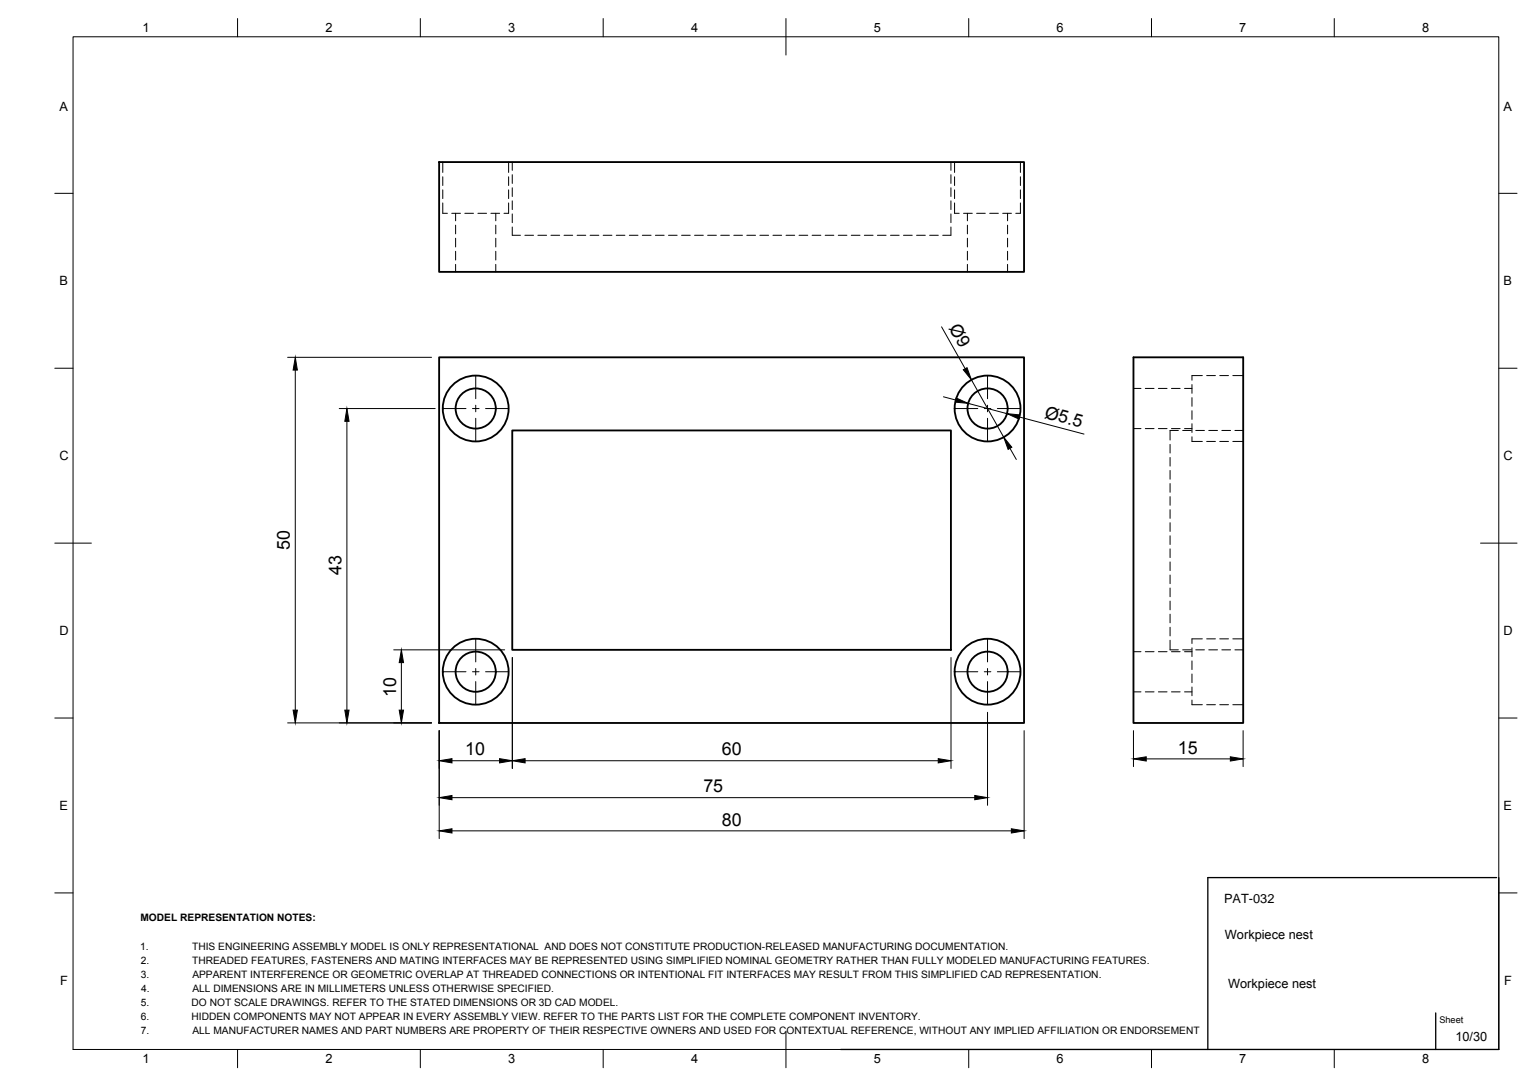
ISO-10303-21;
HEADER;
/* Generated by software containing ST-Developer
 * from STEP Tools, Inc. (www.steptools.com) 
 */

FILE_DESCRIPTION(
/* description */ ('Drill jig with bushing plate'),
/* implementation_level */ '2;1');

FILE_NAME(
/* name */ 'Workpiece nest.step',
/* time_stamp */ '2026-10-27T10:51:08-07:00',
/* author */ (''),
/* organization */ (''),
/* preprocessor_version */ 'ST-DEVELOPER v20.2',
/* originating_system */ 'Autodesk Translation Framework v15.17.0.0',
/* authorisation */ '');

FILE_SCHEMA (('AUTOMOTIVE_DESIGN { 1 0 10303 214 3 1 1 }'));
ENDSEC;

DATA;
#10=MECHANICAL_DESIGN_GEOMETRIC_PRESENTATION_REPRESENTATION('',(#228),#6638);
#180=SHAPE_REPRESENTATION_RELATIONSHIP('SRR','None',#6744,#204);
#204=ADVANCED_BREP_SHAPE_REPRESENTATION('',(#252),#6617);
#228=STYLED_ITEM('',(#6936),#252);
#252=MANIFOLD_SOLID_BREP('Body1',#3595);
#297=FACE_BOUND('',#777,.T.);
#298=FACE_BOUND('',#780,.T.);
#299=FACE_BOUND('',#783,.T.);
#300=FACE_BOUND('',#786,.T.);
#301=FACE_BOUND('',#801,.T.);
#302=FACE_BOUND('',#802,.T.);
#303=FACE_BOUND('',#803,.T.);
#304=FACE_BOUND('',#804,.T.);
#305=FACE_BOUND('',#805,.T.);
#306=FACE_BOUND('',#807,.T.);
#307=FACE_BOUND('',#808,.T.);
#308=FACE_BOUND('',#809,.T.);
#309=FACE_BOUND('',#810,.T.);
#384=PLANE('',#3960);
#385=PLANE('',#3965);
#386=PLANE('',#3970);
#387=PLANE('',#3975);
#388=PLANE('',#3985);
#389=PLANE('',#3986);
#390=PLANE('',#3987);
#391=PLANE('',#3988);
#392=PLANE('',#3989);
#393=PLANE('',#3990);
#394=PLANE('',#3991);
#395=PLANE('',#3992);
#396=PLANE('',#3993);
#397=PLANE('',#3994);
#398=PLANE('',#3995);
#533=FACE_OUTER_BOUND('',#775,.T.);
#534=FACE_OUTER_BOUND('',#776,.T.);
#535=FACE_OUTER_BOUND('',#778,.T.);
#536=FACE_OUTER_BOUND('',#779,.T.);
#537=FACE_OUTER_BOUND('',#781,.T.);
#538=FACE_OUTER_BOUND('',#782,.T.);
#539=FACE_OUTER_BOUND('',#784,.T.);
#540=FACE_OUTER_BOUND('',#785,.T.);
#541=FACE_OUTER_BOUND('',#787,.T.);
#542=FACE_OUTER_BOUND('',#788,.T.);
#543=FACE_OUTER_BOUND('',#789,.T.);
#544=FACE_OUTER_BOUND('',#790,.T.);
#545=FACE_OUTER_BOUND('',#791,.T.);
#546=FACE_OUTER_BOUND('',#792,.T.);
#547=FACE_OUTER_BOUND('',#793,.T.);
#548=FACE_OUTER_BOUND('',#794,.T.);
#549=FACE_OUTER_BOUND('',#795,.T.);
#550=FACE_OUTER_BOUND('',#796,.T.);
#551=FACE_OUTER_BOUND('',#797,.T.);
#552=FACE_OUTER_BOUND('',#798,.T.);
#553=FACE_OUTER_BOUND('',#799,.T.);
#554=FACE_OUTER_BOUND('',#800,.T.);
#555=FACE_OUTER_BOUND('',#806,.T.);
#775=EDGE_LOOP('',(#2569,#2570,#2571,#2572));
#776=EDGE_LOOP('',(#2573));
#777=EDGE_LOOP('',(#2574));
#778=EDGE_LOOP('',(#2575,#2576,#2577,#2578));
#779=EDGE_LOOP('',(#2579));
#780=EDGE_LOOP('',(#2580));
#781=EDGE_LOOP('',(#2581,#2582,#2583,#2584));
#782=EDGE_LOOP('',(#2585));
#783=EDGE_LOOP('',(#2586));
#784=EDGE_LOOP('',(#2587,#2588,#2589,#2590));
#785=EDGE_LOOP('',(#2591));
#786=EDGE_LOOP('',(#2592));
#787=EDGE_LOOP('',(#2593,#2594,#2595,#2596));
#788=EDGE_LOOP('',(#2597,#2598,#2599,#2600));
#789=EDGE_LOOP('',(#2601,#2602,#2603,#2604));
#790=EDGE_LOOP('',(#2605,#2606,#2607,#2608));
#791=EDGE_LOOP('',(#2609,#2610,#2611,#2612));
#792=EDGE_LOOP('',(#2613,#2614,#2615,#2616));
#793=EDGE_LOOP('',(#2617,#2618,#2619,#2620));
#794=EDGE_LOOP('',(#2621,#2622,#2623,#2624));
#795=EDGE_LOOP('',(#2625,#2626,#2627,#2628));
#796=EDGE_LOOP('',(#2629,#2630,#2631,#2632));
#797=EDGE_LOOP('',(#2633,#2634,#2635,#2636));
#798=EDGE_LOOP('',(#2637,#2638,#2639,#2640));
#799=EDGE_LOOP('',(#2641,#2642,#2643,#2644));
#800=EDGE_LOOP('',(#2645,#2646,#2647,#2648));
#801=EDGE_LOOP('',(#2649,#2650,#2651,#2652));
#802=EDGE_LOOP('',(#2653));
#803=EDGE_LOOP('',(#2654));
#804=EDGE_LOOP('',(#2655));
#805=EDGE_LOOP('',(#2656));
#806=EDGE_LOOP('',(#2657,#2658,#2659,#2660));
#807=EDGE_LOOP('',(#2661));
#808=EDGE_LOOP('',(#2662));
#809=EDGE_LOOP('',(#2663));
#810=EDGE_LOOP('',(#2664));
#1060=LINE('',#5640,#1321);
#1061=LINE('',#5649,#1322);
#1062=LINE('',#5658,#1323);
#1063=LINE('',#5667,#1324);
#1064=LINE('',#5675,#1325);
#1065=LINE('',#5679,#1326);
#1066=LINE('',#5683,#1327);
#1067=LINE('',#5687,#1328);
#1068=LINE('',#5691,#1329);
#1069=LINE('',#5693,#1330);
#1070=LINE('',#5695,#1331);
#1071=LINE('',#5696,#1332);
#1072=LINE('',#5699,#1333);
#1073=LINE('',#5701,#1334);
#1074=LINE('',#5702,#1335);
#1075=LINE('',#5705,#1336);
#1076=LINE('',#5707,#1337);
#1077=LINE('',#5708,#1338);
#1078=LINE('',#5710,#1339);
#1079=LINE('',#5711,#1340);
#1080=LINE('',#5716,#1341);
#1081=LINE('',#5718,#1342);
#1082=LINE('',#5720,#1343);
#1083=LINE('',#5721,#1344);
#1084=LINE('',#5724,#1345);
#1085=LINE('',#5726,#1346);
#1086=LINE('',#5727,#1347);
#1087=LINE('',#5730,#1348);
#1088=LINE('',#5732,#1349);
#1089=LINE('',#5733,#1350);
#1090=LINE('',#5735,#1351);
#1091=LINE('',#5736,#1352);
#1321=VECTOR('',#4515,0.45);
#1322=VECTOR('',#4526,0.45);
#1323=VECTOR('',#4537,0.45);
#1324=VECTOR('',#4548,0.45);
#1325=VECTOR('',#4559,0.275);
#1326=VECTOR('',#4564,0.275);
#1327=VECTOR('',#4569,0.275);
#1328=VECTOR('',#4574,0.275);
#1329=VECTOR('',#4577,1.);
#1330=VECTOR('',#4578,1.);
#1331=VECTOR('',#4579,1.);
#1332=VECTOR('',#4580,1.);
#1333=VECTOR('',#4583,1.);
#1334=VECTOR('',#4584,1.);
#1335=VECTOR('',#4585,1.);
#1336=VECTOR('',#4588,1.);
#1337=VECTOR('',#4589,1.);
#1338=VECTOR('',#4590,1.);
#1339=VECTOR('',#4593,1.);
#1340=VECTOR('',#4594,1.);
#1341=VECTOR('',#4599,1.);
#1342=VECTOR('',#4600,1.);
#1343=VECTOR('',#4601,1.);
#1344=VECTOR('',#4602,1.);
#1345=VECTOR('',#4605,1.);
#1346=VECTOR('',#4606,1.);
#1347=VECTOR('',#4607,1.);
#1348=VECTOR('',#4610,1.);
#1349=VECTOR('',#4611,1.);
#1350=VECTOR('',#4612,1.);
#1351=VECTOR('',#4615,1.);
#1352=VECTOR('',#4616,1.);
#1588=CIRCLE('',#3958,0.45);
#1589=CIRCLE('',#3959,0.45);
#1590=CIRCLE('',#3961,0.275);
#1591=CIRCLE('',#3963,0.45);
#1592=CIRCLE('',#3964,0.45);
#1593=CIRCLE('',#3966,0.275);
#1594=CIRCLE('',#3968,0.45);
#1595=CIRCLE('',#3969,0.45);
#1596=CIRCLE('',#3971,0.275);
#1597=CIRCLE('',#3973,0.45);
#1598=CIRCLE('',#3974,0.45);
#1599=CIRCLE('',#3976,0.275);
#1600=CIRCLE('',#3978,0.275);
#1601=CIRCLE('',#3980,0.275);
#1602=CIRCLE('',#3982,0.275);
#1603=CIRCLE('',#3984,0.275);
#1764=VERTEX_POINT('',#5637);
#1765=VERTEX_POINT('',#5639);
#1766=VERTEX_POINT('',#5643);
#1767=VERTEX_POINT('',#5646);
#1768=VERTEX_POINT('',#5648);
#1769=VERTEX_POINT('',#5652);
#1770=VERTEX_POINT('',#5655);
#1771=VERTEX_POINT('',#5657);
#1772=VERTEX_POINT('',#5661);
#1773=VERTEX_POINT('',#5664);
#1774=VERTEX_POINT('',#5666);
#1775=VERTEX_POINT('',#5670);
#1776=VERTEX_POINT('',#5673);
#1777=VERTEX_POINT('',#5677);
#1778=VERTEX_POINT('',#5681);
#1779=VERTEX_POINT('',#5685);
#1780=VERTEX_POINT('',#5689);
#1781=VERTEX_POINT('',#5690);
#1782=VERTEX_POINT('',#5692);
#1783=VERTEX_POINT('',#5694);
#1784=VERTEX_POINT('',#5698);
#1785=VERTEX_POINT('',#5700);
#1786=VERTEX_POINT('',#5704);
#1787=VERTEX_POINT('',#5706);
#1788=VERTEX_POINT('',#5714);
#1789=VERTEX_POINT('',#5715);
#1790=VERTEX_POINT('',#5717);
#1791=VERTEX_POINT('',#5719);
#1792=VERTEX_POINT('',#5723);
#1793=VERTEX_POINT('',#5725);
#1794=VERTEX_POINT('',#5729);
#1795=VERTEX_POINT('',#5731);
#2072=EDGE_CURVE('',#1764,#1764,#1588,.T.);
#2073=EDGE_CURVE('',#1764,#1765,#1060,.T.);
#2074=EDGE_CURVE('',#1765,#1765,#1589,.T.);
#2075=EDGE_CURVE('',#1766,#1766,#1590,.T.);
#2076=EDGE_CURVE('',#1767,#1767,#1591,.T.);
#2077=EDGE_CURVE('',#1767,#1768,#1061,.T.);
#2078=EDGE_CURVE('',#1768,#1768,#1592,.T.);
#2079=EDGE_CURVE('',#1769,#1769,#1593,.T.);
#2080=EDGE_CURVE('',#1770,#1770,#1594,.T.);
#2081=EDGE_CURVE('',#1770,#1771,#1062,.T.);
#2082=EDGE_CURVE('',#1771,#1771,#1595,.T.);
#2083=EDGE_CURVE('',#1772,#1772,#1596,.T.);
#2084=EDGE_CURVE('',#1773,#1773,#1597,.T.);
#2085=EDGE_CURVE('',#1773,#1774,#1063,.T.);
#2086=EDGE_CURVE('',#1774,#1774,#1598,.T.);
#2087=EDGE_CURVE('',#1775,#1775,#1599,.T.);
#2088=EDGE_CURVE('',#1776,#1776,#1600,.T.);
#2089=EDGE_CURVE('',#1776,#1766,#1064,.T.);
#2090=EDGE_CURVE('',#1777,#1777,#1601,.T.);
#2091=EDGE_CURVE('',#1777,#1769,#1065,.T.);
#2092=EDGE_CURVE('',#1778,#1778,#1602,.T.);
#2093=EDGE_CURVE('',#1778,#1772,#1066,.T.);
#2094=EDGE_CURVE('',#1779,#1779,#1603,.T.);
#2095=EDGE_CURVE('',#1779,#1775,#1067,.T.);
#2096=EDGE_CURVE('',#1780,#1781,#1068,.T.);
#2097=EDGE_CURVE('',#1782,#1780,#1069,.T.);
#2098=EDGE_CURVE('',#1783,#1782,#1070,.T.);
#2099=EDGE_CURVE('',#1783,#1781,#1071,.T.);
#2100=EDGE_CURVE('',#1781,#1784,#1072,.T.);
#2101=EDGE_CURVE('',#1785,#1783,#1073,.T.);
#2102=EDGE_CURVE('',#1785,#1784,#1074,.T.);
#2103=EDGE_CURVE('',#1784,#1786,#1075,.T.);
#2104=EDGE_CURVE('',#1787,#1785,#1076,.T.);
#2105=EDGE_CURVE('',#1787,#1786,#1077,.T.);
#2106=EDGE_CURVE('',#1786,#1780,#1078,.T.);
#2107=EDGE_CURVE('',#1782,#1787,#1079,.T.);
#2108=EDGE_CURVE('',#1788,#1789,#1080,.T.);
#2109=EDGE_CURVE('',#1789,#1790,#1081,.T.);
#2110=EDGE_CURVE('',#1791,#1790,#1082,.T.);
#2111=EDGE_CURVE('',#1788,#1791,#1083,.T.);
#2112=EDGE_CURVE('',#1792,#1788,#1084,.T.);
#2113=EDGE_CURVE('',#1793,#1791,#1085,.T.);
#2114=EDGE_CURVE('',#1792,#1793,#1086,.T.);
#2115=EDGE_CURVE('',#1794,#1792,#1087,.T.);
#2116=EDGE_CURVE('',#1795,#1793,#1088,.T.);
#2117=EDGE_CURVE('',#1794,#1795,#1089,.T.);
#2118=EDGE_CURVE('',#1789,#1794,#1090,.T.);
#2119=EDGE_CURVE('',#1790,#1795,#1091,.T.);
#2569=ORIENTED_EDGE('',*,*,#2072,.F.);
#2570=ORIENTED_EDGE('',*,*,#2073,.T.);
#2571=ORIENTED_EDGE('',*,*,#2074,.F.);
#2572=ORIENTED_EDGE('',*,*,#2073,.F.);
#2573=ORIENTED_EDGE('',*,*,#2072,.T.);
#2574=ORIENTED_EDGE('',*,*,#2075,.F.);
#2575=ORIENTED_EDGE('',*,*,#2076,.F.);
#2576=ORIENTED_EDGE('',*,*,#2077,.T.);
#2577=ORIENTED_EDGE('',*,*,#2078,.F.);
#2578=ORIENTED_EDGE('',*,*,#2077,.F.);
#2579=ORIENTED_EDGE('',*,*,#2076,.T.);
#2580=ORIENTED_EDGE('',*,*,#2079,.F.);
#2581=ORIENTED_EDGE('',*,*,#2080,.F.);
#2582=ORIENTED_EDGE('',*,*,#2081,.T.);
#2583=ORIENTED_EDGE('',*,*,#2082,.F.);
#2584=ORIENTED_EDGE('',*,*,#2081,.F.);
#2585=ORIENTED_EDGE('',*,*,#2080,.T.);
#2586=ORIENTED_EDGE('',*,*,#2083,.F.);
#2587=ORIENTED_EDGE('',*,*,#2084,.F.);
#2588=ORIENTED_EDGE('',*,*,#2085,.T.);
#2589=ORIENTED_EDGE('',*,*,#2086,.F.);
#2590=ORIENTED_EDGE('',*,*,#2085,.F.);
#2591=ORIENTED_EDGE('',*,*,#2084,.T.);
#2592=ORIENTED_EDGE('',*,*,#2087,.F.);
#2593=ORIENTED_EDGE('',*,*,#2088,.F.);
#2594=ORIENTED_EDGE('',*,*,#2089,.T.);
#2595=ORIENTED_EDGE('',*,*,#2075,.T.);
#2596=ORIENTED_EDGE('',*,*,#2089,.F.);
#2597=ORIENTED_EDGE('',*,*,#2090,.F.);
#2598=ORIENTED_EDGE('',*,*,#2091,.T.);
#2599=ORIENTED_EDGE('',*,*,#2079,.T.);
#2600=ORIENTED_EDGE('',*,*,#2091,.F.);
#2601=ORIENTED_EDGE('',*,*,#2092,.F.);
#2602=ORIENTED_EDGE('',*,*,#2093,.T.);
#2603=ORIENTED_EDGE('',*,*,#2083,.T.);
#2604=ORIENTED_EDGE('',*,*,#2093,.F.);
#2605=ORIENTED_EDGE('',*,*,#2094,.F.);
#2606=ORIENTED_EDGE('',*,*,#2095,.T.);
#2607=ORIENTED_EDGE('',*,*,#2087,.T.);
#2608=ORIENTED_EDGE('',*,*,#2095,.F.);
#2609=ORIENTED_EDGE('',*,*,#2096,.F.);
#2610=ORIENTED_EDGE('',*,*,#2097,.F.);
#2611=ORIENTED_EDGE('',*,*,#2098,.F.);
#2612=ORIENTED_EDGE('',*,*,#2099,.T.);
#2613=ORIENTED_EDGE('',*,*,#2100,.F.);
#2614=ORIENTED_EDGE('',*,*,#2099,.F.);
#2615=ORIENTED_EDGE('',*,*,#2101,.F.);
#2616=ORIENTED_EDGE('',*,*,#2102,.T.);
#2617=ORIENTED_EDGE('',*,*,#2103,.F.);
#2618=ORIENTED_EDGE('',*,*,#2102,.F.);
#2619=ORIENTED_EDGE('',*,*,#2104,.F.);
#2620=ORIENTED_EDGE('',*,*,#2105,.T.);
#2621=ORIENTED_EDGE('',*,*,#2106,.F.);
#2622=ORIENTED_EDGE('',*,*,#2105,.F.);
#2623=ORIENTED_EDGE('',*,*,#2107,.F.);
#2624=ORIENTED_EDGE('',*,*,#2097,.T.);
#2625=ORIENTED_EDGE('',*,*,#2101,.T.);
#2626=ORIENTED_EDGE('',*,*,#2098,.T.);
#2627=ORIENTED_EDGE('',*,*,#2107,.T.);
#2628=ORIENTED_EDGE('',*,*,#2104,.T.);
#2629=ORIENTED_EDGE('',*,*,#2108,.T.);
#2630=ORIENTED_EDGE('',*,*,#2109,.T.);
#2631=ORIENTED_EDGE('',*,*,#2110,.F.);
#2632=ORIENTED_EDGE('',*,*,#2111,.F.);
#2633=ORIENTED_EDGE('',*,*,#2112,.T.);
#2634=ORIENTED_EDGE('',*,*,#2111,.T.);
#2635=ORIENTED_EDGE('',*,*,#2113,.F.);
#2636=ORIENTED_EDGE('',*,*,#2114,.F.);
#2637=ORIENTED_EDGE('',*,*,#2115,.T.);
#2638=ORIENTED_EDGE('',*,*,#2114,.T.);
#2639=ORIENTED_EDGE('',*,*,#2116,.F.);
#2640=ORIENTED_EDGE('',*,*,#2117,.F.);
#2641=ORIENTED_EDGE('',*,*,#2118,.T.);
#2642=ORIENTED_EDGE('',*,*,#2117,.T.);
#2643=ORIENTED_EDGE('',*,*,#2119,.F.);
#2644=ORIENTED_EDGE('',*,*,#2109,.F.);
#2645=ORIENTED_EDGE('',*,*,#2119,.T.);
#2646=ORIENTED_EDGE('',*,*,#2116,.T.);
#2647=ORIENTED_EDGE('',*,*,#2113,.T.);
#2648=ORIENTED_EDGE('',*,*,#2110,.T.);
#2649=ORIENTED_EDGE('',*,*,#2103,.T.);
#2650=ORIENTED_EDGE('',*,*,#2106,.T.);
#2651=ORIENTED_EDGE('',*,*,#2096,.T.);
#2652=ORIENTED_EDGE('',*,*,#2100,.T.);
#2653=ORIENTED_EDGE('',*,*,#2086,.T.);
#2654=ORIENTED_EDGE('',*,*,#2082,.T.);
#2655=ORIENTED_EDGE('',*,*,#2078,.T.);
#2656=ORIENTED_EDGE('',*,*,#2074,.T.);
#2657=ORIENTED_EDGE('',*,*,#2118,.F.);
#2658=ORIENTED_EDGE('',*,*,#2108,.F.);
#2659=ORIENTED_EDGE('',*,*,#2112,.F.);
#2660=ORIENTED_EDGE('',*,*,#2115,.F.);
#2661=ORIENTED_EDGE('',*,*,#2088,.T.);
#2662=ORIENTED_EDGE('',*,*,#2090,.T.);
#2663=ORIENTED_EDGE('',*,*,#2092,.T.);
#2664=ORIENTED_EDGE('',*,*,#2094,.T.);
#3317=CYLINDRICAL_SURFACE('',#3957,0.45);
#3318=CYLINDRICAL_SURFACE('',#3962,0.45);
#3319=CYLINDRICAL_SURFACE('',#3967,0.45);
#3320=CYLINDRICAL_SURFACE('',#3972,0.45);
#3321=CYLINDRICAL_SURFACE('',#3977,0.275);
#3322=CYLINDRICAL_SURFACE('',#3979,0.275);
#3323=CYLINDRICAL_SURFACE('',#3981,0.275);
#3324=CYLINDRICAL_SURFACE('',#3983,0.275);
#3408=ADVANCED_FACE('',(#533),#3317,.F.);
#3409=ADVANCED_FACE('',(#534,#297),#384,.T.);
#3410=ADVANCED_FACE('',(#535),#3318,.F.);
#3411=ADVANCED_FACE('',(#536,#298),#385,.T.);
#3412=ADVANCED_FACE('',(#537),#3319,.F.);
#3413=ADVANCED_FACE('',(#538,#299),#386,.T.);
#3414=ADVANCED_FACE('',(#539),#3320,.F.);
#3415=ADVANCED_FACE('',(#540,#300),#387,.T.);
#3416=ADVANCED_FACE('',(#541),#3321,.F.);
#3417=ADVANCED_FACE('',(#542),#3322,.F.);
#3418=ADVANCED_FACE('',(#543),#3323,.F.);
#3419=ADVANCED_FACE('',(#544),#3324,.F.);
#3420=ADVANCED_FACE('',(#545),#388,.F.);
#3421=ADVANCED_FACE('',(#546),#389,.F.);
#3422=ADVANCED_FACE('',(#547),#390,.F.);
#3423=ADVANCED_FACE('',(#548),#391,.F.);
#3424=ADVANCED_FACE('',(#549),#392,.T.);
#3425=ADVANCED_FACE('',(#550),#393,.T.);
#3426=ADVANCED_FACE('',(#551),#394,.T.);
#3427=ADVANCED_FACE('',(#552),#395,.T.);
#3428=ADVANCED_FACE('',(#553),#396,.T.);
#3429=ADVANCED_FACE('',(#554,#301,#302,#303,#304,#305),#397,.T.);
#3430=ADVANCED_FACE('',(#555,#306,#307,#308,#309),#398,.F.);
#3595=CLOSED_SHELL('',(#3408,#3409,#3410,#3411,#3412,#3413,#3414,#3415,
#3416,#3417,#3418,#3419,#3420,#3421,#3422,#3423,#3424,#3425,#3426,#3427,
#3428,#3429,#3430));
#3956=AXIS2_PLACEMENT_3D('',#5635,#4509,#4510);
#3957=AXIS2_PLACEMENT_3D('',#5636,#4511,#4512);
#3958=AXIS2_PLACEMENT_3D('',#5638,#4513,#4514);
#3959=AXIS2_PLACEMENT_3D('',#5641,#4516,#4517);
#3960=AXIS2_PLACEMENT_3D('',#5642,#4518,#4519);
#3961=AXIS2_PLACEMENT_3D('',#5644,#4520,#4521);
#3962=AXIS2_PLACEMENT_3D('',#5645,#4522,#4523);
#3963=AXIS2_PLACEMENT_3D('',#5647,#4524,#4525);
#3964=AXIS2_PLACEMENT_3D('',#5650,#4527,#4528);
#3965=AXIS2_PLACEMENT_3D('',#5651,#4529,#4530);
#3966=AXIS2_PLACEMENT_3D('',#5653,#4531,#4532);
#3967=AXIS2_PLACEMENT_3D('',#5654,#4533,#4534);
#3968=AXIS2_PLACEMENT_3D('',#5656,#4535,#4536);
#3969=AXIS2_PLACEMENT_3D('',#5659,#4538,#4539);
#3970=AXIS2_PLACEMENT_3D('',#5660,#4540,#4541);
#3971=AXIS2_PLACEMENT_3D('',#5662,#4542,#4543);
#3972=AXIS2_PLACEMENT_3D('',#5663,#4544,#4545);
#3973=AXIS2_PLACEMENT_3D('',#5665,#4546,#4547);
#3974=AXIS2_PLACEMENT_3D('',#5668,#4549,#4550);
#3975=AXIS2_PLACEMENT_3D('',#5669,#4551,#4552);
#3976=AXIS2_PLACEMENT_3D('',#5671,#4553,#4554);
#3977=AXIS2_PLACEMENT_3D('',#5672,#4555,#4556);
#3978=AXIS2_PLACEMENT_3D('',#5674,#4557,#4558);
#3979=AXIS2_PLACEMENT_3D('',#5676,#4560,#4561);
#3980=AXIS2_PLACEMENT_3D('',#5678,#4562,#4563);
#3981=AXIS2_PLACEMENT_3D('',#5680,#4565,#4566);
#3982=AXIS2_PLACEMENT_3D('',#5682,#4567,#4568);
#3983=AXIS2_PLACEMENT_3D('',#5684,#4570,#4571);
#3984=AXIS2_PLACEMENT_3D('',#5686,#4572,#4573);
#3985=AXIS2_PLACEMENT_3D('',#5688,#4575,#4576);
#3986=AXIS2_PLACEMENT_3D('',#5697,#4581,#4582);
#3987=AXIS2_PLACEMENT_3D('',#5703,#4586,#4587);
#3988=AXIS2_PLACEMENT_3D('',#5709,#4591,#4592);
#3989=AXIS2_PLACEMENT_3D('',#5712,#4595,#4596);
#3990=AXIS2_PLACEMENT_3D('',#5713,#4597,#4598);
#3991=AXIS2_PLACEMENT_3D('',#5722,#4603,#4604);
#3992=AXIS2_PLACEMENT_3D('',#5728,#4608,#4609);
#3993=AXIS2_PLACEMENT_3D('',#5734,#4613,#4614);
#3994=AXIS2_PLACEMENT_3D('',#5737,#4617,#4618);
#3995=AXIS2_PLACEMENT_3D('',#5738,#4619,#4620);
#4509=DIRECTION('axis',(0.,0.,1.));
#4510=DIRECTION('refdir',(1.,0.,0.));
#4511=DIRECTION('center_axis',(0.,0.,1.));
#4512=DIRECTION('ref_axis',(1.,0.,0.));
#4513=DIRECTION('center_axis',(0.,0.,1.));
#4514=DIRECTION('ref_axis',(1.,0.,0.));
#4515=DIRECTION('',(0.,0.,1.));
#4516=DIRECTION('center_axis',(0.,0.,-1.));
#4517=DIRECTION('ref_axis',(1.,0.,0.));
#4518=DIRECTION('center_axis',(0.,0.,1.));
#4519=DIRECTION('ref_axis',(1.,0.,0.));
#4520=DIRECTION('center_axis',(0.,0.,1.));
#4521=DIRECTION('ref_axis',(1.,0.,0.));
#4522=DIRECTION('center_axis',(0.,0.,1.));
#4523=DIRECTION('ref_axis',(1.,0.,0.));
#4524=DIRECTION('center_axis',(0.,0.,1.));
#4525=DIRECTION('ref_axis',(1.,0.,0.));
#4526=DIRECTION('',(0.,0.,1.));
#4527=DIRECTION('center_axis',(0.,0.,-1.));
#4528=DIRECTION('ref_axis',(1.,0.,0.));
#4529=DIRECTION('center_axis',(0.,0.,1.));
#4530=DIRECTION('ref_axis',(1.,0.,0.));
#4531=DIRECTION('center_axis',(0.,0.,1.));
#4532=DIRECTION('ref_axis',(1.,0.,0.));
#4533=DIRECTION('center_axis',(0.,0.,1.));
#4534=DIRECTION('ref_axis',(1.,0.,0.));
#4535=DIRECTION('center_axis',(0.,0.,1.));
#4536=DIRECTION('ref_axis',(1.,0.,0.));
#4537=DIRECTION('',(0.,0.,1.));
#4538=DIRECTION('center_axis',(0.,0.,-1.));
#4539=DIRECTION('ref_axis',(1.,0.,0.));
#4540=DIRECTION('center_axis',(0.,0.,1.));
#4541=DIRECTION('ref_axis',(1.,0.,0.));
#4542=DIRECTION('center_axis',(0.,0.,1.));
#4543=DIRECTION('ref_axis',(1.,0.,0.));
#4544=DIRECTION('center_axis',(0.,0.,1.));
#4545=DIRECTION('ref_axis',(1.,0.,0.));
#4546=DIRECTION('center_axis',(0.,0.,1.));
#4547=DIRECTION('ref_axis',(1.,0.,0.));
#4548=DIRECTION('',(0.,0.,1.));
#4549=DIRECTION('center_axis',(0.,0.,-1.));
#4550=DIRECTION('ref_axis',(1.,0.,0.));
#4551=DIRECTION('center_axis',(0.,0.,1.));
#4552=DIRECTION('ref_axis',(1.,0.,0.));
#4553=DIRECTION('center_axis',(0.,0.,1.));
#4554=DIRECTION('ref_axis',(1.,0.,0.));
#4555=DIRECTION('center_axis',(0.,0.,1.));
#4556=DIRECTION('ref_axis',(1.,0.,0.));
#4557=DIRECTION('center_axis',(0.,0.,1.));
#4558=DIRECTION('ref_axis',(1.,0.,0.));
#4559=DIRECTION('',(0.,0.,1.));
#4560=DIRECTION('center_axis',(0.,0.,1.));
#4561=DIRECTION('ref_axis',(1.,0.,0.));
#4562=DIRECTION('center_axis',(0.,0.,1.));
#4563=DIRECTION('ref_axis',(1.,0.,0.));
#4564=DIRECTION('',(0.,0.,1.));
#4565=DIRECTION('center_axis',(0.,0.,1.));
#4566=DIRECTION('ref_axis',(1.,0.,0.));
#4567=DIRECTION('center_axis',(0.,0.,1.));
#4568=DIRECTION('ref_axis',(1.,0.,0.));
#4569=DIRECTION('',(0.,0.,1.));
#4570=DIRECTION('center_axis',(0.,0.,1.));
#4571=DIRECTION('ref_axis',(1.,0.,0.));
#4572=DIRECTION('center_axis',(0.,0.,1.));
#4573=DIRECTION('ref_axis',(1.,0.,0.));
#4574=DIRECTION('',(0.,0.,1.));
#4575=DIRECTION('center_axis',(0.,-1.,0.));
#4576=DIRECTION('ref_axis',(1.,0.,0.));
#4577=DIRECTION('',(-1.,0.,0.));
#4578=DIRECTION('',(0.,0.,1.));
#4579=DIRECTION('',(1.,0.,0.));
#4580=DIRECTION('',(0.,0.,1.));
#4581=DIRECTION('center_axis',(-1.,0.,0.));
#4582=DIRECTION('ref_axis',(0.,-1.,0.));
#4583=DIRECTION('',(0.,1.,0.));
#4584=DIRECTION('',(0.,-1.,0.));
#4585=DIRECTION('',(0.,0.,1.));
#4586=DIRECTION('center_axis',(0.,1.,0.));
#4587=DIRECTION('ref_axis',(-1.,0.,0.));
#4588=DIRECTION('',(1.,0.,0.));
#4589=DIRECTION('',(-1.,0.,0.));
#4590=DIRECTION('',(0.,0.,1.));
#4591=DIRECTION('center_axis',(1.,0.,0.));
#4592=DIRECTION('ref_axis',(0.,1.,0.));
#4593=DIRECTION('',(0.,-1.,0.));
#4594=DIRECTION('',(0.,1.,0.));
#4595=DIRECTION('center_axis',(0.,0.,1.));
#4596=DIRECTION('ref_axis',(1.,0.,0.));
#4597=DIRECTION('center_axis',(0.,1.,0.));
#4598=DIRECTION('ref_axis',(-1.,0.,0.));
#4599=DIRECTION('',(-1.,0.,0.));
#4600=DIRECTION('',(0.,0.,1.));
#4601=DIRECTION('',(-1.,0.,0.));
#4602=DIRECTION('',(0.,0.,1.));
#4603=DIRECTION('center_axis',(1.,0.,0.));
#4604=DIRECTION('ref_axis',(0.,1.,0.));
#4605=DIRECTION('',(0.,1.,0.));
#4606=DIRECTION('',(0.,1.,0.));
#4607=DIRECTION('',(0.,0.,1.));
#4608=DIRECTION('center_axis',(0.,-1.,0.));
#4609=DIRECTION('ref_axis',(1.,0.,0.));
#4610=DIRECTION('',(1.,0.,0.));
#4611=DIRECTION('',(1.,0.,0.));
#4612=DIRECTION('',(0.,0.,1.));
#4613=DIRECTION('center_axis',(-1.,0.,0.));
#4614=DIRECTION('ref_axis',(0.,-1.,0.));
#4615=DIRECTION('',(0.,-1.,0.));
#4616=DIRECTION('',(0.,-1.,0.));
#4617=DIRECTION('center_axis',(0.,0.,1.));
#4618=DIRECTION('ref_axis',(1.,0.,0.));
#4619=DIRECTION('center_axis',(0.,0.,1.));
#4620=DIRECTION('ref_axis',(1.,0.,0.));
#5635=CARTESIAN_POINT('',(0.,0.,0.));
#5636=CARTESIAN_POINT('Origin',(3.5,-1.8,1.8));
#5637=CARTESIAN_POINT('',(3.05,-1.8,1.8));
#5638=CARTESIAN_POINT('Origin',(3.5,-1.8,1.8));
#5639=CARTESIAN_POINT('',(3.05,-1.8,2.5));
#5640=CARTESIAN_POINT('',(3.05,-1.8,1.8));
#5641=CARTESIAN_POINT('Origin',(3.5,-1.8,2.5));
#5642=CARTESIAN_POINT('Origin',(3.5,-1.8,1.8));
#5643=CARTESIAN_POINT('',(3.225,-1.8,1.8));
#5644=CARTESIAN_POINT('Origin',(3.5,-1.8,1.8));
#5645=CARTESIAN_POINT('Origin',(-3.5,1.8,1.8));
#5646=CARTESIAN_POINT('',(-3.95,1.8,1.8));
#5647=CARTESIAN_POINT('Origin',(-3.5,1.8,1.8));
#5648=CARTESIAN_POINT('',(-3.95,1.8,2.5));
#5649=CARTESIAN_POINT('',(-3.95,1.8,1.8));
#5650=CARTESIAN_POINT('Origin',(-3.5,1.8,2.5));
#5651=CARTESIAN_POINT('Origin',(-3.5,1.8,1.8));
#5652=CARTESIAN_POINT('',(-3.775,1.8,1.8));
#5653=CARTESIAN_POINT('Origin',(-3.5,1.8,1.8));
#5654=CARTESIAN_POINT('Origin',(-3.5,-1.8,1.8));
#5655=CARTESIAN_POINT('',(-3.95,-1.8,1.8));
#5656=CARTESIAN_POINT('Origin',(-3.5,-1.8,1.8));
#5657=CARTESIAN_POINT('',(-3.95,-1.8,2.5));
#5658=CARTESIAN_POINT('',(-3.95,-1.8,1.8));
#5659=CARTESIAN_POINT('Origin',(-3.5,-1.8,2.5));
#5660=CARTESIAN_POINT('Origin',(-3.5,-1.8,1.8));
#5661=CARTESIAN_POINT('',(-3.775,-1.8,1.8));
#5662=CARTESIAN_POINT('Origin',(-3.5,-1.8,1.8));
#5663=CARTESIAN_POINT('Origin',(3.5,1.8,1.8));
#5664=CARTESIAN_POINT('',(3.05,1.8,1.8));
#5665=CARTESIAN_POINT('Origin',(3.5,1.8,1.8));
#5666=CARTESIAN_POINT('',(3.05,1.8,2.5));
#5667=CARTESIAN_POINT('',(3.05,1.8,1.8));
#5668=CARTESIAN_POINT('Origin',(3.5,1.8,2.5));
#5669=CARTESIAN_POINT('Origin',(3.5,1.8,1.8));
#5670=CARTESIAN_POINT('',(3.225,1.8,1.8));
#5671=CARTESIAN_POINT('Origin',(3.5,1.8,1.8));
#5672=CARTESIAN_POINT('Origin',(3.5,-1.8,0.9));
#5673=CARTESIAN_POINT('',(3.225,-1.8,1.));
#5674=CARTESIAN_POINT('Origin',(3.5,-1.8,1.));
#5675=CARTESIAN_POINT('',(3.225,-1.8,0.9));
#5676=CARTESIAN_POINT('Origin',(-3.5,1.8,0.9));
#5677=CARTESIAN_POINT('',(-3.775,1.8,1.));
#5678=CARTESIAN_POINT('Origin',(-3.5,1.8,1.));
#5679=CARTESIAN_POINT('',(-3.775,1.8,0.9));
#5680=CARTESIAN_POINT('Origin',(-3.5,-1.8,0.9));
#5681=CARTESIAN_POINT('',(-3.775,-1.8,1.));
#5682=CARTESIAN_POINT('Origin',(-3.5,-1.8,1.));
#5683=CARTESIAN_POINT('',(-3.775,-1.8,0.9));
#5684=CARTESIAN_POINT('Origin',(3.5,1.8,0.9));
#5685=CARTESIAN_POINT('',(3.225,1.8,1.));
#5686=CARTESIAN_POINT('Origin',(3.5,1.8,1.));
#5687=CARTESIAN_POINT('',(3.225,1.8,0.9));
#5688=CARTESIAN_POINT('Origin',(-3.,-1.5,1.5));
#5689=CARTESIAN_POINT('',(3.,-1.5,2.5));
#5690=CARTESIAN_POINT('',(-3.,-1.5,2.5));
#5691=CARTESIAN_POINT('',(-1.5,-1.5,2.5));
#5692=CARTESIAN_POINT('',(3.,-1.5,1.5));
#5693=CARTESIAN_POINT('',(3.,-1.5,1.5));
#5694=CARTESIAN_POINT('',(-3.,-1.5,1.5));
#5695=CARTESIAN_POINT('',(-3.,-1.5,1.5));
#5696=CARTESIAN_POINT('',(-3.,-1.5,1.5));
#5697=CARTESIAN_POINT('Origin',(-3.,1.5,1.5));
#5698=CARTESIAN_POINT('',(-3.,1.5,2.5));
#5699=CARTESIAN_POINT('',(-3.,0.75,2.5));
#5700=CARTESIAN_POINT('',(-3.,1.5,1.5));
#5701=CARTESIAN_POINT('',(-3.,1.5,1.5));
#5702=CARTESIAN_POINT('',(-3.,1.5,1.5));
#5703=CARTESIAN_POINT('Origin',(3.,1.5,1.5));
#5704=CARTESIAN_POINT('',(3.,1.5,2.5));
#5705=CARTESIAN_POINT('',(1.5,1.5,2.5));
#5706=CARTESIAN_POINT('',(3.,1.5,1.5));
#5707=CARTESIAN_POINT('',(3.,1.5,1.5));
#5708=CARTESIAN_POINT('',(3.,1.5,1.5));
#5709=CARTESIAN_POINT('Origin',(3.,-1.5,1.5));
#5710=CARTESIAN_POINT('',(3.,-0.75,2.5));
#5711=CARTESIAN_POINT('',(3.,-1.5,1.5));
#5712=CARTESIAN_POINT('Origin',(0.,0.,1.5));
#5713=CARTESIAN_POINT('Origin',(4.,2.5,1.));
#5714=CARTESIAN_POINT('',(4.,2.5,1.));
#5715=CARTESIAN_POINT('',(-4.,2.5,1.));
#5716=CARTESIAN_POINT('',(4.,2.5,1.));
#5717=CARTESIAN_POINT('',(-4.,2.5,2.5));
#5718=CARTESIAN_POINT('',(-4.,2.5,1.));
#5719=CARTESIAN_POINT('',(4.,2.5,2.5));
#5720=CARTESIAN_POINT('',(4.,2.5,2.5));
#5721=CARTESIAN_POINT('',(4.,2.5,1.));
#5722=CARTESIAN_POINT('Origin',(4.,-2.5,1.));
#5723=CARTESIAN_POINT('',(4.,-2.5,1.));
#5724=CARTESIAN_POINT('',(4.,-2.5,1.));
#5725=CARTESIAN_POINT('',(4.,-2.5,2.5));
#5726=CARTESIAN_POINT('',(4.,-2.5,2.5));
#5727=CARTESIAN_POINT('',(4.,-2.5,1.));
#5728=CARTESIAN_POINT('Origin',(-4.,-2.5,1.));
#5729=CARTESIAN_POINT('',(-4.,-2.5,1.));
#5730=CARTESIAN_POINT('',(-4.,-2.5,1.));
#5731=CARTESIAN_POINT('',(-4.,-2.5,2.5));
#5732=CARTESIAN_POINT('',(-4.,-2.5,2.5));
#5733=CARTESIAN_POINT('',(-4.,-2.5,1.));
#5734=CARTESIAN_POINT('Origin',(-4.,2.5,1.));
#5735=CARTESIAN_POINT('',(-4.,2.5,1.));
#5736=CARTESIAN_POINT('',(-4.,2.5,2.5));
#5737=CARTESIAN_POINT('Origin',(0.,0.,2.5));
#5738=CARTESIAN_POINT('Origin',(0.,0.,1.));
#6588=UNCERTAINTY_MEASURE_WITH_UNIT(LENGTH_MEASURE(0.001),#6639,
'DISTANCE_ACCURACY_VALUE',
'Maximum model space distance between geometric entities at asserted c
onnectivities');
#6609=UNCERTAINTY_MEASURE_WITH_UNIT(LENGTH_MEASURE(0.001),#6639,
'DISTANCE_ACCURACY_VALUE',
'Maximum model space distance between geometric entities at asserted c
onnectivities');
#6617=(
GEOMETRIC_REPRESENTATION_CONTEXT(3)
GLOBAL_UNCERTAINTY_ASSIGNED_CONTEXT((#6588))
GLOBAL_UNIT_ASSIGNED_CONTEXT((#6639,#6641,#6642))
REPRESENTATION_CONTEXT('','3D')
);
#6638=(
GEOMETRIC_REPRESENTATION_CONTEXT(3)
GLOBAL_UNCERTAINTY_ASSIGNED_CONTEXT((#6609))
GLOBAL_UNIT_ASSIGNED_CONTEXT((#6639,#6641,#6642))
REPRESENTATION_CONTEXT('','3D')
);
#6639=(
LENGTH_UNIT()
NAMED_UNIT(*)
SI_UNIT(.CENTI.,.METRE.)
);
#6641=(
NAMED_UNIT(*)
PLANE_ANGLE_UNIT()
SI_UNIT($,.RADIAN.)
);
#6642=(
NAMED_UNIT(*)
SI_UNIT($,.STERADIAN.)
SOLID_ANGLE_UNIT()
);
#6650=SHAPE_DEFINITION_REPRESENTATION(#6678,#6744);
#6678=PRODUCT_DEFINITION_SHAPE('',$,#6773);
#6744=SHAPE_REPRESENTATION('',(#3956),#6617);
#6765=PRODUCT_DEFINITION_CONTEXT('part definition',#6851,'design');
#6773=PRODUCT_DEFINITION('Workpiece nest','Workpiece nest',#6801,#6765);
#6801=PRODUCT_DEFINITION_FORMATION('',$,#6860);
#6851=APPLICATION_CONTEXT(
'Core Data for Automotive Mechanical Design Process');
#6852=PRODUCT_CONTEXT('part definition',#6851,'mechanical');
#6860=PRODUCT('Workpiece nest','Workpiece nest','Workpiece nest',(#6852));
#6930=COLOUR_RGB('Sky Blue',0.24,0.69,0.87);
#6931=FILL_AREA_STYLE_COLOUR('',#6930);
#6932=FILL_AREA_STYLE('',(#6931));
#6933=SURFACE_STYLE_FILL_AREA(#6932);
#6934=SURFACE_SIDE_STYLE('',(#6933));
#6935=SURFACE_STYLE_USAGE(.BOTH.,#6934);
#6936=PRESENTATION_STYLE_ASSIGNMENT((#6935));
ENDSEC;
END-ISO-10303-21;
